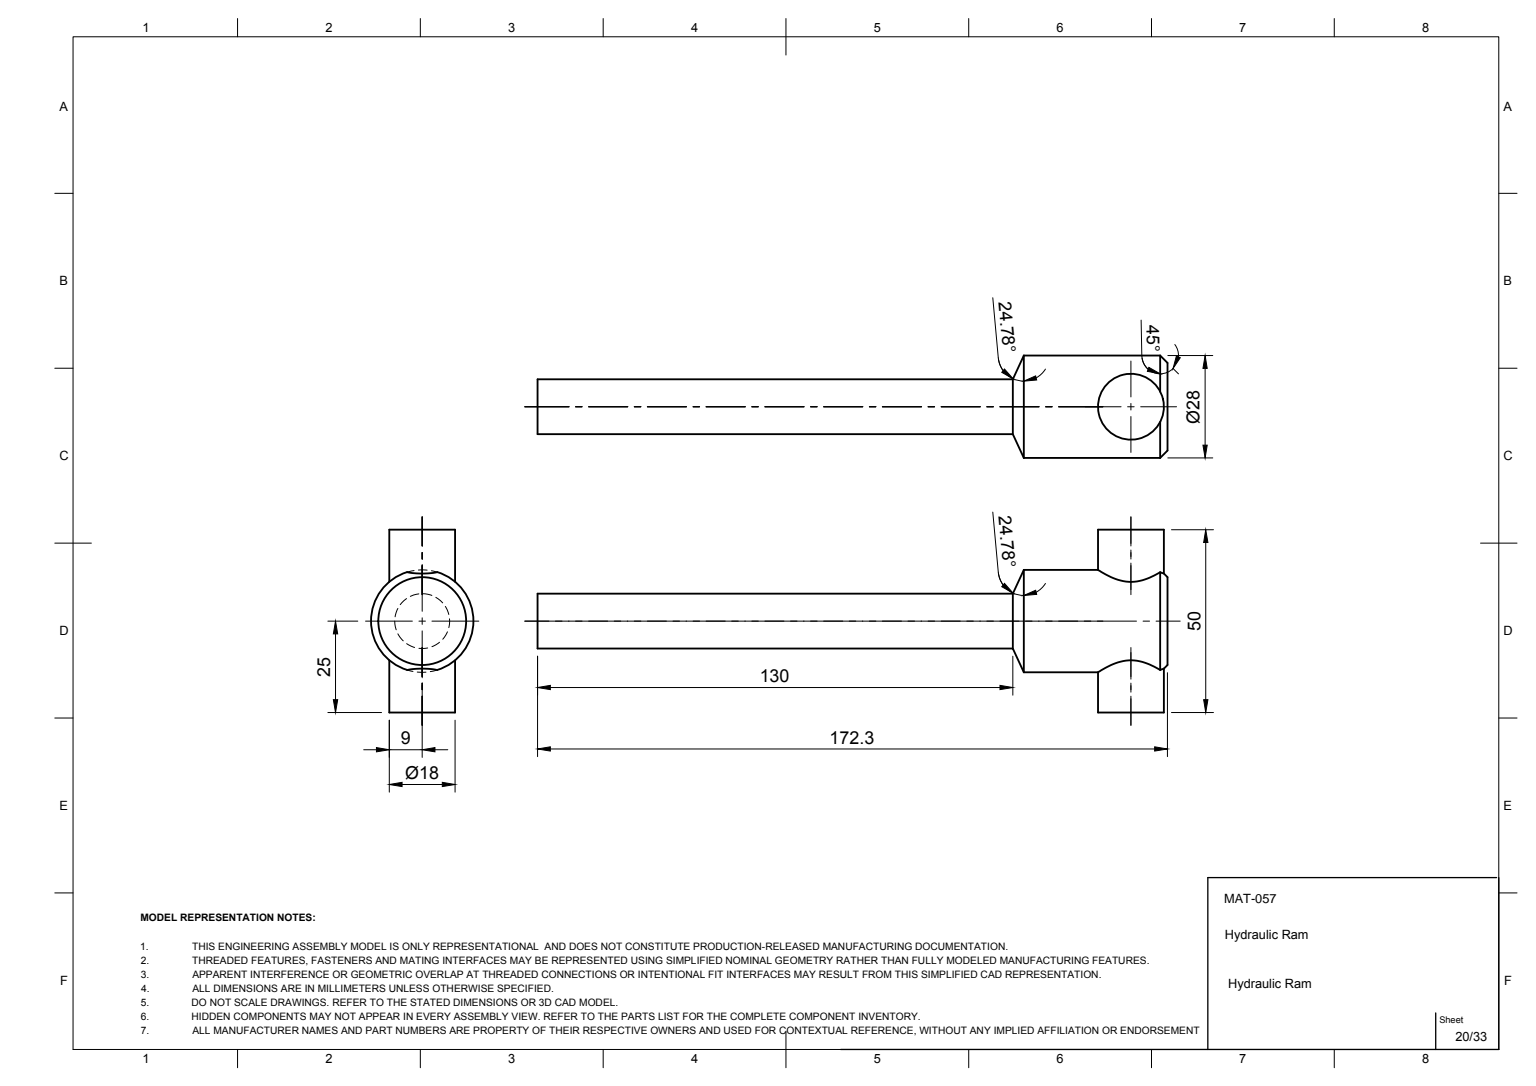
ISO-10303-21;
HEADER;
/* Generated by software containing ST-Developer
 * from STEP Tools, Inc. (www.steptools.com) 
 */

FILE_DESCRIPTION(
/* description */ ('STEP AP214', 'CAx-IF Rec.Pracs.---Representation and Presentation of Product Manufa
cturing Information (PMI)---4.0---2014-10-13'),
/* implementation_level */ '2;1');

FILE_NAME(
/* name */ 'Hydraulic Ram.step',
/* time_stamp */ '2026-10-28T23:34:22+01:00',
/* author */ (''),
/* organization */ (''),
/* preprocessor_version */ 'ST-DEVELOPER v20.2',
/* originating_system */ 'Autodesk Translation Framework v15.17.0.0',
/* authorisation */ '');

FILE_SCHEMA (('AP242_MANAGED_MODEL_BASED_3D_ENGINEERING_MIM_LF { 1 0 10303 442 2 1 4 }'));
ENDSEC;

DATA;
#10=MECHANICAL_DESIGN_GEOMETRIC_PRESENTATION_REPRESENTATION('',(#260),#27807);
#214=SHAPE_REPRESENTATION_RELATIONSHIP('SRR','None',#27911,#236);
#236=ADVANCED_BREP_SHAPE_REPRESENTATION('',(#289),#27791);
#260=STYLED_ITEM('',(#28070),#289);
#289=MANIFOLD_SOLID_BREP('Body1',#12036);
#635=PLANE('',#13182);
#636=PLANE('',#13183);
#637=PLANE('',#13184);
#638=PLANE('',#13185);
#898=B_SPLINE_CURVE_WITH_KNOTS('',3,(#21135,#21136,#21137,#21138,#21139,
#21140,#21141,#21142,#21143,#21144),.UNSPECIFIED.,.F.,.F.,(4,2,2,2,4),(-1.46797143552028,
-1.30470040394833,-1.06055016507708,-0.816399926205828,-0.65312889463391),
 .UNSPECIFIED.);
#899=B_SPLINE_CURVE_WITH_KNOTS('',3,(#21152,#21153,#21154,#21155,#21156,
#21157,#21158,#21159,#21160,#21161),.UNSPECIFIED.,.F.,.F.,(4,2,2,2,4),(0.653128894633879,
0.816399926205827,1.06055016507708,1.30470040394833,1.46797143552025),
 .UNSPECIFIED.);
#900=B_SPLINE_CURVE_WITH_KNOTS('',3,(#21164,#21165,#21166,#21167,#21168,
#21169,#21170,#21171,#21172,#21173,#21174,#21175,#21176,#21177,#21178,#21179),
 .UNSPECIFIED.,.F.,.F.,(4,2,2,2,2,2,2,4),(1.82537904839244,2.10770426762789,
2.46113598680775,2.81456770598761,3.16799942516747,3.52143114434733,3.87164135166438,
4.22185155898142),.UNSPECIFIED.);
#901=B_SPLINE_CURVE_WITH_KNOTS('',3,(#21183,#21184,#21185,#21186,#21187,
#21188,#21189,#21190,#21191,#21192,#21193,#21194,#21195,#21196,#21197,#21198,
#21199),.UNSPECIFIED.,.F.,.F.,(4,2,2,2,3,2,2,4),(4.22185155898142,4.57206176629846,
4.92227197361551,5.27570369279537,5.62913541197523,5.98256713115509,6.33599885033495,
6.61832406957041),.UNSPECIFIED.);
#902=B_SPLINE_CURVE_WITH_KNOTS('',3,(#21205,#21206,#21207,#21208,#21209,
#21210,#21211,#21212,#21213,#21214,#21215,#21216,#21217,#21218,#21219,#21220),
 .UNSPECIFIED.,.F.,.F.,(4,2,2,2,2,2,2,4),(1.40728385299381,1.75749406031085,
2.10770426762789,2.46113598680775,2.81456770598761,3.16799942516747,3.52143114434734,
3.8037563635828),.UNSPECIFIED.);
#903=B_SPLINE_CURVE_WITH_KNOTS('',3,(#21221,#21222,#21223,#21224,#21225,
#21226,#21227,#21228,#21229,#21230,#21231,#21232,#21233,#21234,#21235,#21236,
#21237),.UNSPECIFIED.,.F.,.F.,(4,2,2,3,2,2,2,4),(-0.989188657595171,-0.706863438359723,
-0.353431719179861,8.88178419700125E-16,0.353431719179861,0.706863438359721,
1.05707364567676,1.40728385299381),.UNSPECIFIED.);
#1132=CYLINDRICAL_SURFACE('',#13170,9.00000000000001);
#1133=CYLINDRICAL_SURFACE('',#13172,9.00000000000001);
#1134=CYLINDRICAL_SURFACE('',#13179,7.50000000000001);
#1135=CYLINDRICAL_SURFACE('',#13181,14.);
#1654=FACE_OUTER_BOUND('',#2426,.T.);
#1655=FACE_OUTER_BOUND('',#2427,.T.);
#1656=FACE_OUTER_BOUND('',#2428,.T.);
#1657=FACE_OUTER_BOUND('',#2429,.T.);
#1658=FACE_OUTER_BOUND('',#2430,.T.);
#1659=FACE_OUTER_BOUND('',#2431,.T.);
#1660=FACE_OUTER_BOUND('',#2432,.T.);
#1661=FACE_OUTER_BOUND('',#2433,.T.);
#1662=FACE_OUTER_BOUND('',#2434,.T.);
#1663=FACE_OUTER_BOUND('',#2435,.T.);
#2426=EDGE_LOOP('',(#9915,#9916,#9917,#9918,#9919,#9920,#9921,#9922));
#2427=EDGE_LOOP('',(#9923,#9924,#9925,#9926,#9927,#9928));
#2428=EDGE_LOOP('',(#9929,#9930,#9931,#9932,#9933,#9934));
#2429=EDGE_LOOP('',(#9935,#9936,#9937,#9938,#9939,#9940));
#2430=EDGE_LOOP('',(#9941,#9942,#9943,#9944,#9945));
#2431=EDGE_LOOP('',(#9946,#9947,#9948,#9949,#9950,#9951,#9952,#9953,#9954,
#9955,#9956));
#2432=EDGE_LOOP('',(#9957));
#2433=EDGE_LOOP('',(#9958));
#2434=EDGE_LOOP('',(#9959));
#2435=EDGE_LOOP('',(#9960));
#3269=LINE('',#21148,#4089);
#3270=LINE('',#21181,#4090);
#3271=LINE('',#21204,#4091);
#3272=LINE('',#21243,#4092);
#3273=LINE('',#21251,#4093);
#3274=LINE('',#21253,#4094);
#4089=VECTOR('',#15987,14.);
#4090=VECTOR('',#15994,9.00000000000001);
#4091=VECTOR('',#16001,9.00000000000001);
#4092=VECTOR('',#16006,7.50000000000001);
#4093=VECTOR('',#16017,7.50000000000001);
#4094=VECTOR('',#16020,14.);
#4790=CIRCLE('',#13166,14.);
#4791=CIRCLE('',#13167,14.);
#4792=CIRCLE('',#13168,12.);
#4793=CIRCLE('',#13169,14.);
#4794=CIRCLE('',#13171,9.00000000000001);
#4795=CIRCLE('',#13173,9.00000000000001);
#4796=CIRCLE('',#13175,14.);
#4797=CIRCLE('',#13176,7.50000000000001);
#4798=CIRCLE('',#13177,7.50000000000001);
#4799=CIRCLE('',#13178,14.);
#4800=CIRCLE('',#13180,7.50000000000001);
#5699=VERTEX_POINT('',#21131);
#5700=VERTEX_POINT('',#21132);
#5701=VERTEX_POINT('',#21134);
#5702=VERTEX_POINT('',#21145);
#5703=VERTEX_POINT('',#21147);
#5704=VERTEX_POINT('',#21150);
#5705=VERTEX_POINT('',#21163);
#5706=VERTEX_POINT('',#21180);
#5707=VERTEX_POINT('',#21201);
#5708=VERTEX_POINT('',#21203);
#5709=VERTEX_POINT('',#21239);
#5710=VERTEX_POINT('',#21240);
#5711=VERTEX_POINT('',#21242);
#5712=VERTEX_POINT('',#21244);
#5713=VERTEX_POINT('',#21249);
#7170=EDGE_CURVE('',#5699,#5700,#4790,.T.);
#7171=EDGE_CURVE('',#5701,#5699,#898,.F.);
#7172=EDGE_CURVE('',#5702,#5701,#4791,.T.);
#7173=EDGE_CURVE('',#5702,#5703,#3269,.T.);
#7174=EDGE_CURVE('',#5703,#5703,#4792,.T.);
#7175=EDGE_CURVE('',#5704,#5702,#4793,.T.);
#7176=EDGE_CURVE('',#5700,#5704,#899,.F.);
#7177=EDGE_CURVE('',#5705,#5704,#900,.F.);
#7178=EDGE_CURVE('',#5705,#5706,#3270,.T.);
#7179=EDGE_CURVE('',#5706,#5706,#4794,.T.);
#7180=EDGE_CURVE('',#5700,#5705,#901,.F.);
#7181=EDGE_CURVE('',#5707,#5707,#4795,.T.);
#7182=EDGE_CURVE('',#5707,#5708,#3271,.T.);
#7183=EDGE_CURVE('',#5701,#5708,#902,.F.);
#7184=EDGE_CURVE('',#5708,#5699,#903,.F.);
#7185=EDGE_CURVE('',#5709,#5710,#4796,.T.);
#7186=EDGE_CURVE('',#5710,#5711,#3272,.T.);
#7187=EDGE_CURVE('',#5711,#5712,#4797,.T.);
#7188=EDGE_CURVE('',#5712,#5711,#4798,.T.);
#7189=EDGE_CURVE('',#5710,#5709,#4799,.T.);
#7190=EDGE_CURVE('',#5713,#5713,#4800,.T.);
#7191=EDGE_CURVE('',#5713,#5712,#3273,.T.);
#7192=EDGE_CURVE('',#5709,#5702,#3274,.T.);
#9915=ORIENTED_EDGE('',*,*,#7170,.F.);
#9916=ORIENTED_EDGE('',*,*,#7171,.F.);
#9917=ORIENTED_EDGE('',*,*,#7172,.F.);
#9918=ORIENTED_EDGE('',*,*,#7173,.T.);
#9919=ORIENTED_EDGE('',*,*,#7174,.F.);
#9920=ORIENTED_EDGE('',*,*,#7173,.F.);
#9921=ORIENTED_EDGE('',*,*,#7175,.F.);
#9922=ORIENTED_EDGE('',*,*,#7176,.F.);
#9923=ORIENTED_EDGE('',*,*,#7176,.T.);
#9924=ORIENTED_EDGE('',*,*,#7177,.F.);
#9925=ORIENTED_EDGE('',*,*,#7178,.T.);
#9926=ORIENTED_EDGE('',*,*,#7179,.F.);
#9927=ORIENTED_EDGE('',*,*,#7178,.F.);
#9928=ORIENTED_EDGE('',*,*,#7180,.F.);
#9929=ORIENTED_EDGE('',*,*,#7181,.T.);
#9930=ORIENTED_EDGE('',*,*,#7182,.T.);
#9931=ORIENTED_EDGE('',*,*,#7183,.F.);
#9932=ORIENTED_EDGE('',*,*,#7171,.T.);
#9933=ORIENTED_EDGE('',*,*,#7184,.F.);
#9934=ORIENTED_EDGE('',*,*,#7182,.F.);
#9935=ORIENTED_EDGE('',*,*,#7185,.T.);
#9936=ORIENTED_EDGE('',*,*,#7186,.T.);
#9937=ORIENTED_EDGE('',*,*,#7187,.T.);
#9938=ORIENTED_EDGE('',*,*,#7188,.T.);
#9939=ORIENTED_EDGE('',*,*,#7186,.F.);
#9940=ORIENTED_EDGE('',*,*,#7189,.T.);
#9941=ORIENTED_EDGE('',*,*,#7190,.T.);
#9942=ORIENTED_EDGE('',*,*,#7191,.T.);
#9943=ORIENTED_EDGE('',*,*,#7187,.F.);
#9944=ORIENTED_EDGE('',*,*,#7188,.F.);
#9945=ORIENTED_EDGE('',*,*,#7191,.F.);
#9946=ORIENTED_EDGE('',*,*,#7185,.F.);
#9947=ORIENTED_EDGE('',*,*,#7192,.T.);
#9948=ORIENTED_EDGE('',*,*,#7172,.T.);
#9949=ORIENTED_EDGE('',*,*,#7183,.T.);
#9950=ORIENTED_EDGE('',*,*,#7184,.T.);
#9951=ORIENTED_EDGE('',*,*,#7170,.T.);
#9952=ORIENTED_EDGE('',*,*,#7180,.T.);
#9953=ORIENTED_EDGE('',*,*,#7177,.T.);
#9954=ORIENTED_EDGE('',*,*,#7175,.T.);
#9955=ORIENTED_EDGE('',*,*,#7192,.F.);
#9956=ORIENTED_EDGE('',*,*,#7189,.F.);
#9957=ORIENTED_EDGE('',*,*,#7190,.F.);
#9958=ORIENTED_EDGE('',*,*,#7174,.T.);
#9959=ORIENTED_EDGE('',*,*,#7181,.F.);
#9960=ORIENTED_EDGE('',*,*,#7179,.T.);
#11306=CONICAL_SURFACE('',#13165,14.,0.785398163397448);
#11307=CONICAL_SURFACE('',#13174,7.50000000000001,1.13838855122436);
#11736=ADVANCED_FACE('',(#1654),#11306,.T.);
#11737=ADVANCED_FACE('',(#1655),#1132,.T.);
#11738=ADVANCED_FACE('',(#1656),#1133,.T.);
#11739=ADVANCED_FACE('',(#1657),#11307,.T.);
#11740=ADVANCED_FACE('',(#1658),#1134,.T.);
#11741=ADVANCED_FACE('',(#1659),#1135,.T.);
#11742=ADVANCED_FACE('',(#1660),#635,.F.);
#11743=ADVANCED_FACE('',(#1661),#636,.T.);
#11744=ADVANCED_FACE('',(#1662),#637,.F.);
#11745=ADVANCED_FACE('',(#1663),#638,.T.);
#12036=CLOSED_SHELL('',(#11736,#11737,#11738,#11739,#11740,#11741,#11742,
#11743,#11744,#11745));
#13164=AXIS2_PLACEMENT_3D('',#21129,#15979,#15980);
#13165=AXIS2_PLACEMENT_3D('',#21130,#15981,#15982);
#13166=AXIS2_PLACEMENT_3D('',#21133,#15983,#15984);
#13167=AXIS2_PLACEMENT_3D('',#21146,#15985,#15986);
#13168=AXIS2_PLACEMENT_3D('',#21149,#15988,#15989);
#13169=AXIS2_PLACEMENT_3D('',#21151,#15990,#15991);
#13170=AXIS2_PLACEMENT_3D('',#21162,#15992,#15993);
#13171=AXIS2_PLACEMENT_3D('',#21182,#15995,#15996);
#13172=AXIS2_PLACEMENT_3D('',#21200,#15997,#15998);
#13173=AXIS2_PLACEMENT_3D('',#21202,#15999,#16000);
#13174=AXIS2_PLACEMENT_3D('',#21238,#16002,#16003);
#13175=AXIS2_PLACEMENT_3D('',#21241,#16004,#16005);
#13176=AXIS2_PLACEMENT_3D('',#21245,#16007,#16008);
#13177=AXIS2_PLACEMENT_3D('',#21246,#16009,#16010);
#13178=AXIS2_PLACEMENT_3D('',#21247,#16011,#16012);
#13179=AXIS2_PLACEMENT_3D('',#21248,#16013,#16014);
#13180=AXIS2_PLACEMENT_3D('',#21250,#16015,#16016);
#13181=AXIS2_PLACEMENT_3D('',#21252,#16018,#16019);
#13182=AXIS2_PLACEMENT_3D('',#21254,#16021,#16022);
#13183=AXIS2_PLACEMENT_3D('',#21255,#16023,#16024);
#13184=AXIS2_PLACEMENT_3D('',#21256,#16025,#16026);
#13185=AXIS2_PLACEMENT_3D('',#21257,#16027,#16028);
#15979=DIRECTION('axis',(0.,0.,1.));
#15980=DIRECTION('refdir',(1.,0.,0.));
#15981=DIRECTION('center_axis',(0.974431531646231,-0.224684645967589,-3.15685775282419E-17));
#15982=DIRECTION('ref_axis',(-0.224684645967589,-0.974431531646231,7.70371977754894E-33));
#15983=DIRECTION('center_axis',(0.974431531646231,-0.224684645967589,-3.15685775282419E-17));
#15984=DIRECTION('ref_axis',(0.224684645967589,0.974431531646231,-7.70371977754894E-33));
#15985=DIRECTION('center_axis',(0.974431531646231,-0.224684645967589,-3.15685775282419E-17));
#15986=DIRECTION('ref_axis',(0.224684645967589,0.974431531646231,3.96508223080413E-15));
#15987=DIRECTION('',(-0.847903180621224,-0.530151107036863,-6.42732503809162E-17));
#15988=DIRECTION('center_axis',(-0.974431531646231,0.224684645967589,3.15685775282419E-17));
#15989=DIRECTION('ref_axis',(0.224684645967589,0.974431531646231,1.00148357108136E-32));
#15990=DIRECTION('center_axis',(0.974431531646231,-0.224684645967589,-3.15685775282419E-17));
#15991=DIRECTION('ref_axis',(0.224684645967589,0.974431531646231,3.96508223080413E-15));
#15992=DIRECTION('center_axis',(1.41649888995139E-16,-4.54281045584161E-17,
1.));
#15993=DIRECTION('ref_axis',(-0.974431531646231,0.224684645967588,1.48235115880738E-16));
#15994=DIRECTION('',(-1.41649888995139E-16,4.54281045584162E-17,-1.));
#15995=DIRECTION('center_axis',(-1.41649888995139E-16,4.54281045584161E-17,
-1.));
#15996=DIRECTION('ref_axis',(0.974431531646231,-0.224684645967588,-1.48235115880738E-16));
#15997=DIRECTION('center_axis',(1.41649888995139E-16,-4.54281045584161E-17,
1.));
#15998=DIRECTION('ref_axis',(-0.974431531646231,0.224684645967588,1.48235115880738E-16));
#15999=DIRECTION('center_axis',(-1.41649888995139E-16,4.54281045584161E-17,
-1.));
#16000=DIRECTION('ref_axis',(0.974431531646231,-0.224684645967588,-1.48235115880738E-16));
#16001=DIRECTION('',(-1.41649888995139E-16,4.54281045584162E-17,-1.));
#16002=DIRECTION('center_axis',(-0.974431531646231,0.224684645967589,3.15685775282419E-17));
#16003=DIRECTION('ref_axis',(0.224684645967589,0.974431531646231,1.00148357108136E-32));
#16004=DIRECTION('center_axis',(0.974431531646231,-0.224684645967589,-3.15685775282419E-17));
#16005=DIRECTION('ref_axis',(-0.224684645967589,-0.974431531646231,7.70371977754894E-33));
#16006=DIRECTION('',(0.612348034572362,0.790588315468528,-1.24422025962473E-16));
#16007=DIRECTION('center_axis',(-0.974431531646231,0.224684645967589,3.15685775282419E-17));
#16008=DIRECTION('ref_axis',(-3.07614173527375E-17,7.09297466563341E-18,
-1.));
#16009=DIRECTION('center_axis',(-0.974431531646231,0.224684645967589,3.15685775282419E-17));
#16010=DIRECTION('ref_axis',(-3.07614173527375E-17,7.09297466563341E-18,
-1.));
#16011=DIRECTION('center_axis',(0.974431531646231,-0.224684645967589,-3.15685775282419E-17));
#16012=DIRECTION('ref_axis',(-0.224684645967589,-0.974431531646231,7.70371977754894E-33));
#16013=DIRECTION('center_axis',(0.974431531646231,-0.224684645967589,-3.15685775282419E-17));
#16014=DIRECTION('ref_axis',(3.07614173527375E-17,-7.09297466563341E-18,
1.));
#16015=DIRECTION('center_axis',(-0.974431531646231,0.224684645967589,3.15685775282419E-17));
#16016=DIRECTION('ref_axis',(-3.07614173527375E-17,7.09297466563341E-18,
-1.));
#16017=DIRECTION('',(-0.974431531646231,0.224684645967589,3.15685775282419E-17));
#16018=DIRECTION('center_axis',(0.974431531646231,-0.224684645967589,-3.15685775282419E-17));
#16019=DIRECTION('ref_axis',(-0.224684645967589,-0.974431531646231,7.70371977754894E-33));
#16020=DIRECTION('',(-0.974431531646231,0.224684645967589,3.15685775282419E-17));
#16021=DIRECTION('center_axis',(-0.974431531646231,0.224684645967589,1.48235115880738E-16));
#16022=DIRECTION('ref_axis',(-1.41649888995139E-16,4.54281045584161E-17,
-1.));
#16023=DIRECTION('center_axis',(-0.974431531646231,0.224684645967589,3.15685775282419E-17));
#16024=DIRECTION('ref_axis',(0.224684645967589,0.974431531646231,3.23381123402325E-17));
#16025=DIRECTION('center_axis',(-2.79663353364523E-17,1.92149246924214E-17,
-1.));
#16026=DIRECTION('ref_axis',(0.974431531646231,-0.224684645967589,-3.15685775282419E-17));
#16027=DIRECTION('center_axis',(-2.79663353364523E-17,1.92149246924214E-17,
-1.));
#16028=DIRECTION('ref_axis',(0.974431531646231,-0.224684645967589,-3.15685775282419E-17));
#21129=CARTESIAN_POINT('',(0.,0.,0.));
#21130=CARTESIAN_POINT('Origin',(35.8297426794921,134.358342876286,253.073593133703));
#21131=CARTESIAN_POINT('',(34.9033441517125,130.340658746376,266.452681293963));
#21132=CARTESIAN_POINT('',(34.9033441517133,130.340658746376,239.694504973444));
#21133=CARTESIAN_POINT('Origin',(35.8297426794921,134.358342876286,253.073593133703));
#21134=CARTESIAN_POINT('',(36.756141207271,138.376027006196,266.452681293963));
#21135=CARTESIAN_POINT('Ctrl Pts',(34.9033441517134,130.340658746376,266.452681293963));
#21136=CARTESIAN_POINT('Ctrl Pts',(34.7662765826152,130.87911435207,266.338527474787));
#21137=CARTESIAN_POINT('Ctrl Pts',(34.6744566711603,131.454679427698,266.253801129437));
#21138=CARTESIAN_POINT('Ctrl Pts',(34.5897191635504,132.90588139296,266.106625474983));
#21139=CARTESIAN_POINT('Ctrl Pts',(34.672455114567,133.79000188487,266.073593133703));
#21140=CARTESIAN_POINT('Ctrl Pts',(35.0381671811249,135.376053159637,266.073593133703));
#21141=CARTESIAN_POINT('Ctrl Pts',(35.3509231135055,136.207135591509,266.106625474983));
#21142=CARTESIAN_POINT('Ctrl Pts',(36.0625567285284,137.474710120736,266.253801129437));
#21143=CARTESIAN_POINT('Ctrl Pts',(36.3971341252449,137.951956407289,266.338527474787));
#21144=CARTESIAN_POINT('Ctrl Pts',(36.756141207271,138.376027006196,266.452681293963));
#21145=CARTESIAN_POINT('',(38.9753277230386,148.000384319333,253.073593133703));
#21146=CARTESIAN_POINT('Origin',(35.8297426794921,134.358342876286,253.073593133703));
#21147=CARTESIAN_POINT('',(36.5770953678107,146.500890547976,253.073593133703));
#21148=CARTESIAN_POINT('',(38.9753277230384,148.000384319333,253.073593133703));
#21149=CARTESIAN_POINT('Origin',(33.8808796161997,134.807712168221,253.073593133703));
#21150=CARTESIAN_POINT('',(36.7561412072705,138.376027006196,239.694504973443));
#21151=CARTESIAN_POINT('Origin',(35.8297426794921,134.358342876286,253.073593133703));
#21152=CARTESIAN_POINT('Ctrl Pts',(36.7561412072712,138.376027006196,239.694504973444));
#21153=CARTESIAN_POINT('Ctrl Pts',(36.397134125245,137.951956407289,239.808658792619));
#21154=CARTESIAN_POINT('Ctrl Pts',(36.0625567285284,137.474710120736,239.893385137969));
#21155=CARTESIAN_POINT('Ctrl Pts',(35.3509231135055,136.207135591509,240.040560792424));
#21156=CARTESIAN_POINT('Ctrl Pts',(35.0381671811249,135.376053159637,240.073593133703));
#21157=CARTESIAN_POINT('Ctrl Pts',(34.672455114567,133.79000188487,240.073593133703));
#21158=CARTESIAN_POINT('Ctrl Pts',(34.5897191635504,132.90588139296,240.040560792424));
#21159=CARTESIAN_POINT('Ctrl Pts',(34.6744566711603,131.454679427698,239.893385137969));
#21160=CARTESIAN_POINT('Ctrl Pts',(34.7662765826152,130.87911435207,239.808658792619));
#21161=CARTESIAN_POINT('Ctrl Pts',(34.9033441517133,130.340658746376,239.694504973444));
#21162=CARTESIAN_POINT('Origin',(43.625194932662,132.560865708545,228.073593133703));
#21163=CARTESIAN_POINT('',(52.3950787174781,130.538703894837,239.073593133703));
#21164=CARTESIAN_POINT('Ctrl Pts',(36.7561412072711,138.376027006196,239.694504973444));
#21165=CARTESIAN_POINT('Ctrl Pts',(37.3757148123747,139.107887080655,239.957180175221));
#21166=CARTESIAN_POINT('Ctrl Pts',(38.1032632208345,139.722699664096,240.284186300941));
#21167=CARTESIAN_POINT('Ctrl Pts',(39.7934459051052,140.779485676509,241.003527112932));
#21168=CARTESIAN_POINT('Ctrl Pts',(40.9089819966417,141.223731124707,241.45444414134));
#21169=CARTESIAN_POINT('Ctrl Pts',(43.2595652384548,141.632211467481,242.135542680051));
#21170=CARTESIAN_POINT('Ctrl Pts',(44.499373374861,141.595451762353,242.34978783894));
#21171=CARTESIAN_POINT('Ctrl Pts',(46.7953401178796,141.066047224369,242.34978783894));
#21172=CARTESIAN_POINT('Ctrl Pts',(47.9260656397772,140.556208735091,242.135542680051));
#21173=CARTESIAN_POINT('Ctrl Pts',(49.8604537880171,139.159698706815,241.45444414134));
#21174=CARTESIAN_POINT('Ctrl Pts',(50.6688322158806,138.271836607652,241.003527112932));
#21175=CARTESIAN_POINT('Ctrl Pts',(51.8384599473883,136.401179241243,240.207376376427));
#21176=CARTESIAN_POINT('Ctrl Pts',(52.2870155925865,135.282886966942,239.801293920092));
#21177=CARTESIAN_POINT('Ctrl Pts',(52.6974998422104,132.921179650313,239.231941806271));
#21178=CARTESIAN_POINT('Ctrl Pts',(52.6573682389623,131.676223457217,239.073593133703));
#21179=CARTESIAN_POINT('Ctrl Pts',(52.3950787174781,130.538703894837,239.073593133703));
#21180=CARTESIAN_POINT('',(52.3950787174781,130.538703894837,228.073593133703));
#21181=CARTESIAN_POINT('',(52.3950787174781,130.538703894837,228.073593133703));
#21182=CARTESIAN_POINT('Origin',(43.625194932662,132.560865708545,228.073593133703));
#21183=CARTESIAN_POINT('Ctrl Pts',(52.3950787174781,130.538703894837,239.073593133703));
#21184=CARTESIAN_POINT('Ctrl Pts',(52.1327891959939,129.401184332456,239.073593133703));
#21185=CARTESIAN_POINT('Ctrl Pts',(51.6237279274457,128.264354049093,239.231941806271));
#21186=CARTESIAN_POINT('Ctrl Pts',(50.2205453140278,126.32084245355,239.801293920092));
#21187=CARTESIAN_POINT('Ctrl Pts',(49.3276013266274,125.511873472089,240.207376376427));
#21188=CARTESIAN_POINT('Ctrl Pts',(47.4569439602189,124.342245740582,241.003527112932));
#21189=CARTESIAN_POINT('Ctrl Pts',(46.3414078686823,123.898000292383,241.45444414134));
#21190=CARTESIAN_POINT('Ctrl Pts',(43.9908246268693,123.489519949609,242.135542680051));
#21191=CARTESIAN_POINT('Ctrl Pts',(42.751016490463,123.526279654737,242.34978783894));
#21192=CARTESIAN_POINT('Ctrl Pts',(41.6030331189537,123.790981923729,242.34978783894));
#21193=CARTESIAN_POINT('Ctrl Pts',(40.4550497474444,124.055684192721,242.34978783894));
#21194=CARTESIAN_POINT('Ctrl Pts',(39.3243242255468,124.565522682,242.135542680051));
#21195=CARTESIAN_POINT('Ctrl Pts',(37.3899360773069,125.962032710275,241.45444414134));
#21196=CARTESIAN_POINT('Ctrl Pts',(36.5815576494434,126.849894809438,241.003527112932));
#21197=CARTESIAN_POINT('Ctrl Pts',(35.5247716370308,128.540077493709,240.284186300941));
#21198=CARTESIAN_POINT('Ctrl Pts',(35.1398950505134,129.411393287529,239.957180175221));
#21199=CARTESIAN_POINT('Ctrl Pts',(34.9033441517133,130.340658746376,239.694504973444));
#21200=CARTESIAN_POINT('Origin',(43.625194932662,132.560865708545,228.073593133703));
#21201=CARTESIAN_POINT('',(52.3950787174781,130.538703894837,278.073593133703));
#21202=CARTESIAN_POINT('Origin',(43.625194932662,132.560865708545,278.073593133703));
#21203=CARTESIAN_POINT('',(52.3950787174781,130.538703894837,267.073593133703));
#21204=CARTESIAN_POINT('',(52.3950787174781,130.538703894837,228.073593133703));
#21205=CARTESIAN_POINT('Ctrl Pts',(52.3950787174781,130.538703894837,267.073593133703));
#21206=CARTESIAN_POINT('Ctrl Pts',(52.6573682389623,131.676223457217,267.073593133703));
#21207=CARTESIAN_POINT('Ctrl Pts',(52.6974998422104,132.921179650313,266.915244461136));
#21208=CARTESIAN_POINT('Ctrl Pts',(52.2870155925865,135.282886966942,266.345892347314));
#21209=CARTESIAN_POINT('Ctrl Pts',(51.8384599473883,136.401179241243,265.939809890979));
#21210=CARTESIAN_POINT('Ctrl Pts',(50.6688322158806,138.271836607652,265.143659154474));
#21211=CARTESIAN_POINT('Ctrl Pts',(49.8604537880171,139.159698706815,264.692742126067));
#21212=CARTESIAN_POINT('Ctrl Pts',(47.9260656397772,140.556208735091,264.011643587355));
#21213=CARTESIAN_POINT('Ctrl Pts',(46.7953401178796,141.066047224369,263.797398428467));
#21214=CARTESIAN_POINT('Ctrl Pts',(44.499373374861,141.595451762353,263.797398428467));
#21215=CARTESIAN_POINT('Ctrl Pts',(43.2595652384548,141.632211467481,264.011643587355));
#21216=CARTESIAN_POINT('Ctrl Pts',(40.9089819966417,141.223731124707,264.692742126067));
#21217=CARTESIAN_POINT('Ctrl Pts',(39.7934459051052,140.779485676509,265.143659154474));
#21218=CARTESIAN_POINT('Ctrl Pts',(38.1032632208345,139.722699664096,265.862999966466));
#21219=CARTESIAN_POINT('Ctrl Pts',(37.3757148123746,139.107887080655,266.190006092186));
#21220=CARTESIAN_POINT('Ctrl Pts',(36.756141207271,138.376027006196,266.452681293963));
#21221=CARTESIAN_POINT('Ctrl Pts',(34.9033441517133,130.340658746376,266.452681293963));
#21222=CARTESIAN_POINT('Ctrl Pts',(35.1398950505135,129.411393287529,266.190006092186));
#21223=CARTESIAN_POINT('Ctrl Pts',(35.5247716370309,128.540077493709,265.862999966466));
#21224=CARTESIAN_POINT('Ctrl Pts',(36.5815576494434,126.849894809438,265.143659154474));
#21225=CARTESIAN_POINT('Ctrl Pts',(37.389936077307,125.962032710275,264.692742126067));
#21226=CARTESIAN_POINT('Ctrl Pts',(39.3243242255468,124.565522682,264.011643587355));
#21227=CARTESIAN_POINT('Ctrl Pts',(40.4550497474444,124.055684192721,263.797398428467));
#21228=CARTESIAN_POINT('Ctrl Pts',(41.6030331189537,123.790981923729,263.797398428467));
#21229=CARTESIAN_POINT('Ctrl Pts',(42.751016490463,123.526279654737,263.797398428467));
#21230=CARTESIAN_POINT('Ctrl Pts',(43.9908246268693,123.489519949609,264.011643587355));
#21231=CARTESIAN_POINT('Ctrl Pts',(46.3414078686823,123.898000292383,264.692742126067));
#21232=CARTESIAN_POINT('Ctrl Pts',(47.4569439602189,124.342245740582,265.143659154474));
#21233=CARTESIAN_POINT('Ctrl Pts',(49.3276013266274,125.511873472089,265.939809890979));
#21234=CARTESIAN_POINT('Ctrl Pts',(50.2205453140278,126.32084245355,266.345892347314));
#21235=CARTESIAN_POINT('Ctrl Pts',(51.6237279274458,128.264354049093,266.915244461136));
#21236=CARTESIAN_POINT('Ctrl Pts',(52.1327891959939,129.401184332456,267.073593133703));
#21237=CARTESIAN_POINT('Ctrl Pts',(52.3950787174781,130.538703894837,267.073593133703));
#21238=CARTESIAN_POINT('Origin',(75.0993334048352,125.303551643792,253.073593133703));
#21239=CARTESIAN_POINT('',(75.3216238534428,139.619647024742,253.073593133703));
#21240=CARTESIAN_POINT('',(69.0304537663503,112.335564138647,253.073593133703));
#21241=CARTESIAN_POINT('Origin',(72.1760388098966,125.977605581695,253.073593133703));
#21242=CARTESIAN_POINT('',(73.4141985600783,117.995315156445,253.073593133703));
#21243=CARTESIAN_POINT('',(73.4141985600783,117.995315156445,253.073593133703));
#21244=CARTESIAN_POINT('',(75.0993334048352,125.303551643792,245.573593133703));
#21245=CARTESIAN_POINT('Origin',(75.0993334048352,125.303551643792,253.073593133703));
#21246=CARTESIAN_POINT('Origin',(75.0993334048352,125.303551643792,253.073593133703));
#21247=CARTESIAN_POINT('Origin',(72.1760388098966,125.977605581695,253.073593133703));
#21248=CARTESIAN_POINT('Origin',(75.0993334048352,125.303551643792,253.073593133703));
#21249=CARTESIAN_POINT('',(201.775432518845,96.0945476680054,245.573593133703));
#21250=CARTESIAN_POINT('Origin',(201.775432518845,96.0945476680054,253.073593133703));
#21251=CARTESIAN_POINT('',(75.0993334048352,125.303551643792,245.573593133703));
#21252=CARTESIAN_POINT('Origin',(75.0993334048352,125.303551643792,253.073593133703));
#21253=CARTESIAN_POINT('',(78.2449184483815,138.945593086839,253.073593133703));
#21254=CARTESIAN_POINT('Origin',(201.775432518845,96.0945476680054,253.073593133703));
#21255=CARTESIAN_POINT('Origin',(33.8808796161997,134.807712168221,253.073593133703));
#21256=CARTESIAN_POINT('Origin',(43.625194932662,132.560865708545,278.073593133703));
#21257=CARTESIAN_POINT('Origin',(43.625194932662,132.560865708545,228.073593133703));
#27762=UNCERTAINTY_MEASURE_WITH_UNIT(LENGTH_MEASURE(0.01),#27808,
'DISTANCE_ACCURACY_VALUE',
'Maximum model space distance between geometric entities at asserted c
onnectivities');
#27778=UNCERTAINTY_MEASURE_WITH_UNIT(LENGTH_MEASURE(0.01),#27808,
'DISTANCE_ACCURACY_VALUE',
'Maximum model space distance between geometric entities at asserted c
onnectivities');
#27791=(
GEOMETRIC_REPRESENTATION_CONTEXT(3)
GLOBAL_UNCERTAINTY_ASSIGNED_CONTEXT((#27762))
GLOBAL_UNIT_ASSIGNED_CONTEXT((#27808,#27810,#27811))
REPRESENTATION_CONTEXT('','3D')
);
#27807=(
GEOMETRIC_REPRESENTATION_CONTEXT(3)
GLOBAL_UNCERTAINTY_ASSIGNED_CONTEXT((#27778))
GLOBAL_UNIT_ASSIGNED_CONTEXT((#27808,#27810,#27811))
REPRESENTATION_CONTEXT('','3D')
);
#27808=(
LENGTH_UNIT()
NAMED_UNIT(*)
SI_UNIT(.MILLI.,.METRE.)
);
#27810=(
NAMED_UNIT(*)
PLANE_ANGLE_UNIT()
SI_UNIT($,.RADIAN.)
);
#27811=(
NAMED_UNIT(*)
SI_UNIT($,.STERADIAN.)
SOLID_ANGLE_UNIT()
);
#27824=SHAPE_DEFINITION_REPRESENTATION(#27857,#27911);
#27857=PRODUCT_DEFINITION_SHAPE('',$,#27940);
#27911=SHAPE_REPRESENTATION('',(#13164),#27791);
#27927=PRODUCT_DEFINITION_CONTEXT('part definition',#28013,'design');
#27940=PRODUCT_DEFINITION('Hydraulic Ram','Hydraulic Ram',#27968,#27927);
#27968=PRODUCT_DEFINITION_FORMATION('',$,#28027);
#28013=APPLICATION_CONTEXT('Managed model based 3d engineering');
#28014=PRODUCT_CONTEXT('part definition',#28013,'mechanical');
#28027=PRODUCT('Hydraulic Ram','Hydraulic Ram',$,(#28014));
#28064=COLOUR_RGB('Sky Blue',0.24,0.69,0.87);
#28065=FILL_AREA_STYLE_COLOUR('',#28064);
#28066=FILL_AREA_STYLE('',(#28065));
#28067=SURFACE_STYLE_FILL_AREA(#28066);
#28068=SURFACE_SIDE_STYLE('',(#28067));
#28069=SURFACE_STYLE_USAGE(.BOTH.,#28068);
#28070=PRESENTATION_STYLE_ASSIGNMENT((#28069));
ENDSEC;
END-ISO-10303-21;
